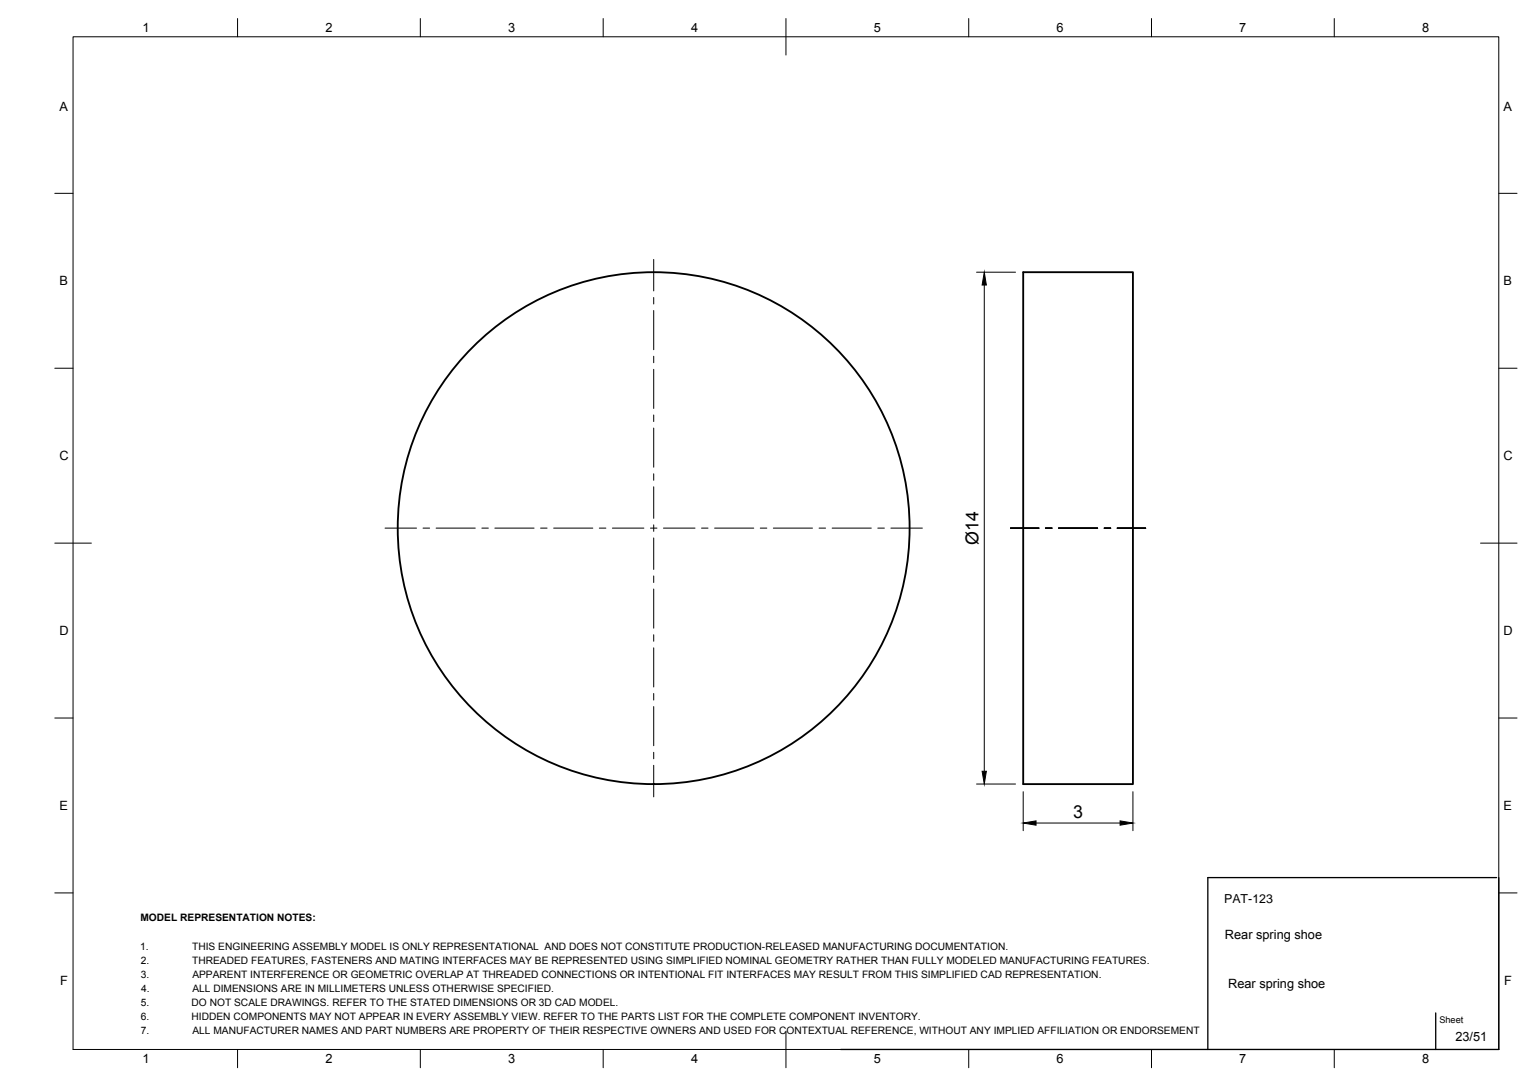
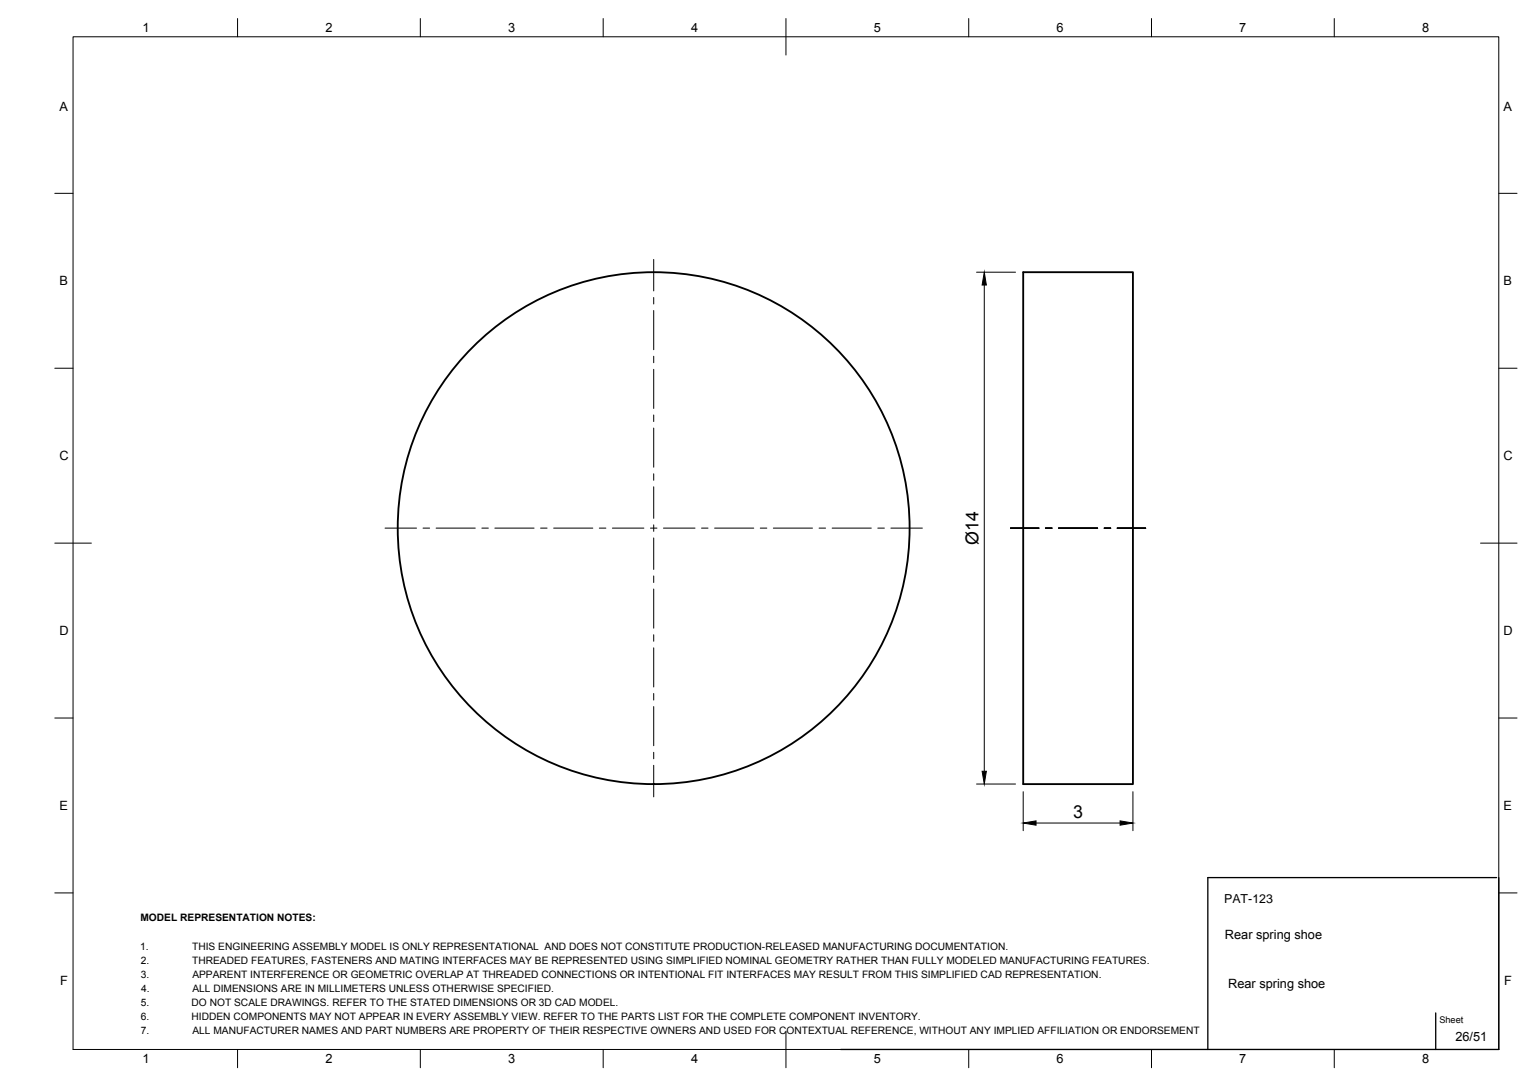
ISO-10303-21;
HEADER;
/* Generated by software containing ST-Developer
 * from STEP Tools, Inc. (www.steptools.com) 
 */

FILE_DESCRIPTION(
/* description */ ('Worm-less right-angle friction wheel drive'),
/* implementation_level */ '2;1');

FILE_NAME(
/* name */ 'Rear spring shoe.step',
/* time_stamp */ '2026-10-28T03:22:36-07:00',
/* author */ (''),
/* organization */ (''),
/* preprocessor_version */ 'ST-DEVELOPER v20.2',
/* originating_system */ 'Autodesk Translation Framework v15.17.0.0',
/* authorisation */ '');

FILE_SCHEMA (('AUTOMOTIVE_DESIGN { 1 0 10303 214 3 1 1 }'));
ENDSEC;

DATA;
#10=MECHANICAL_DESIGN_GEOMETRIC_PRESENTATION_REPRESENTATION('',(#629),#17046);
#535=SHAPE_REPRESENTATION_RELATIONSHIP('SRR','None',#17278,#582);
#582=ADVANCED_BREP_SHAPE_REPRESENTATION('',(#683),#17014);
#629=STYLED_ITEM('',(#17591),#683);
#683=MANIFOLD_SOLID_BREP('Body1',#8184);
#1058=PLANE('',#9211);
#1059=PLANE('',#9212);
#1427=FACE_OUTER_BOUND('',#2083,.T.);
#1428=FACE_OUTER_BOUND('',#2084,.T.);
#1429=FACE_OUTER_BOUND('',#2085,.T.);
#2083=EDGE_LOOP('',(#6572,#6573,#6574,#6575));
#2084=EDGE_LOOP('',(#6576));
#2085=EDGE_LOOP('',(#6577));
#2670=LINE('',#13484,#3210);
#3210=VECTOR('',#11002,0.7);
#3683=CIRCLE('',#9209,0.7);
#3684=CIRCLE('',#9210,0.7);
#4215=VERTEX_POINT('',#13481);
#4216=VERTEX_POINT('',#13483);
#5055=EDGE_CURVE('',#4215,#4215,#3683,.T.);
#5056=EDGE_CURVE('',#4215,#4216,#2670,.T.);
#5057=EDGE_CURVE('',#4216,#4216,#3684,.T.);
#6572=ORIENTED_EDGE('',*,*,#5055,.F.);
#6573=ORIENTED_EDGE('',*,*,#5056,.T.);
#6574=ORIENTED_EDGE('',*,*,#5057,.T.);
#6575=ORIENTED_EDGE('',*,*,#5056,.F.);
#6576=ORIENTED_EDGE('',*,*,#5055,.T.);
#6577=ORIENTED_EDGE('',*,*,#5057,.F.);
#7643=CYLINDRICAL_SURFACE('',#9208,0.7);
#7919=ADVANCED_FACE('',(#1427),#7643,.T.);
#7920=ADVANCED_FACE('',(#1428),#1058,.T.);
#7921=ADVANCED_FACE('',(#1429),#1059,.F.);
#8184=CLOSED_SHELL('',(#7919,#7920,#7921));
#9207=AXIS2_PLACEMENT_3D('',#13479,#10996,#10997);
#9208=AXIS2_PLACEMENT_3D('',#13480,#10998,#10999);
#9209=AXIS2_PLACEMENT_3D('',#13482,#11000,#11001);
#9210=AXIS2_PLACEMENT_3D('',#13485,#11003,#11004);
#9211=AXIS2_PLACEMENT_3D('',#13486,#11005,#11006);
#9212=AXIS2_PLACEMENT_3D('',#13487,#11007,#11008);
#10996=DIRECTION('axis',(0.,0.,1.));
#10997=DIRECTION('refdir',(1.,0.,0.));
#10998=DIRECTION('center_axis',(0.,1.,0.));
#10999=DIRECTION('ref_axis',(1.,0.,0.));
#11000=DIRECTION('center_axis',(0.,1.,0.));
#11001=DIRECTION('ref_axis',(1.,0.,0.));
#11002=DIRECTION('',(0.,-1.,0.));
#11003=DIRECTION('center_axis',(0.,1.,0.));
#11004=DIRECTION('ref_axis',(1.,0.,0.));
#11005=DIRECTION('center_axis',(0.,1.,0.));
#11006=DIRECTION('ref_axis',(1.,0.,0.));
#11007=DIRECTION('center_axis',(0.,1.,0.));
#11008=DIRECTION('ref_axis',(1.,0.,0.));
#13479=CARTESIAN_POINT('',(0.,0.,0.));
#13480=CARTESIAN_POINT('Origin',(-0.3,7.1,4.));
#13481=CARTESIAN_POINT('',(-1.,7.4,4.));
#13482=CARTESIAN_POINT('Origin',(-0.3,7.4,4.));
#13483=CARTESIAN_POINT('',(-1.,7.1,4.));
#13484=CARTESIAN_POINT('',(-1.,7.1,4.));
#13485=CARTESIAN_POINT('Origin',(-0.3,7.1,4.));
#13486=CARTESIAN_POINT('Origin',(-0.3,7.4,4.));
#13487=CARTESIAN_POINT('Origin',(-0.3,7.1,4.));
#16961=UNCERTAINTY_MEASURE_WITH_UNIT(LENGTH_MEASURE(0.001),#17047,
'DISTANCE_ACCURACY_VALUE',
'Maximum model space distance between geometric entities at asserted c
onnectivities');
#16993=UNCERTAINTY_MEASURE_WITH_UNIT(LENGTH_MEASURE(0.001),#17047,
'DISTANCE_ACCURACY_VALUE',
'Maximum model space distance between geometric entities at asserted c
onnectivities');
#17014=(
GEOMETRIC_REPRESENTATION_CONTEXT(3)
GLOBAL_UNCERTAINTY_ASSIGNED_CONTEXT((#16961))
GLOBAL_UNIT_ASSIGNED_CONTEXT((#17047,#17049,#17050))
REPRESENTATION_CONTEXT('','3D')
);
#17046=(
GEOMETRIC_REPRESENTATION_CONTEXT(3)
GLOBAL_UNCERTAINTY_ASSIGNED_CONTEXT((#16993))
GLOBAL_UNIT_ASSIGNED_CONTEXT((#17047,#17049,#17050))
REPRESENTATION_CONTEXT('','3D')
);
#17047=(
LENGTH_UNIT()
NAMED_UNIT(*)
SI_UNIT(.CENTI.,.METRE.)
);
#17049=(
NAMED_UNIT(*)
PLANE_ANGLE_UNIT()
SI_UNIT($,.RADIAN.)
);
#17050=(
NAMED_UNIT(*)
SI_UNIT($,.STERADIAN.)
SOLID_ANGLE_UNIT()
);
#17071=SHAPE_DEFINITION_REPRESENTATION(#17123,#17278);
#17123=PRODUCT_DEFINITION_SHAPE('',$,#17331);
#17278=SHAPE_REPRESENTATION('',(#9207),#17014);
#17310=PRODUCT_DEFINITION_CONTEXT('part definition',#17468,'design');
#17331=PRODUCT_DEFINITION('Rear spring shoe','Rear spring shoe',#17383,
#17310);
#17383=PRODUCT_DEFINITION_FORMATION('',$,#17490);
#17468=APPLICATION_CONTEXT(
'Core Data for Automotive Mechanical Design Process');
#17469=PRODUCT_CONTEXT('part definition',#17468,'mechanical');
#17490=PRODUCT('Rear spring shoe','Rear spring shoe','Rear spring shoe',
(#17469));
#17585=COLOUR_RGB('Grey',0.48,0.52,0.57);
#17586=FILL_AREA_STYLE_COLOUR('',#17585);
#17587=FILL_AREA_STYLE('',(#17586));
#17588=SURFACE_STYLE_FILL_AREA(#17587);
#17589=SURFACE_SIDE_STYLE('',(#17588));
#17590=SURFACE_STYLE_USAGE(.BOTH.,#17589);
#17591=PRESENTATION_STYLE_ASSIGNMENT((#17590));
ENDSEC;
END-ISO-10303-21;
